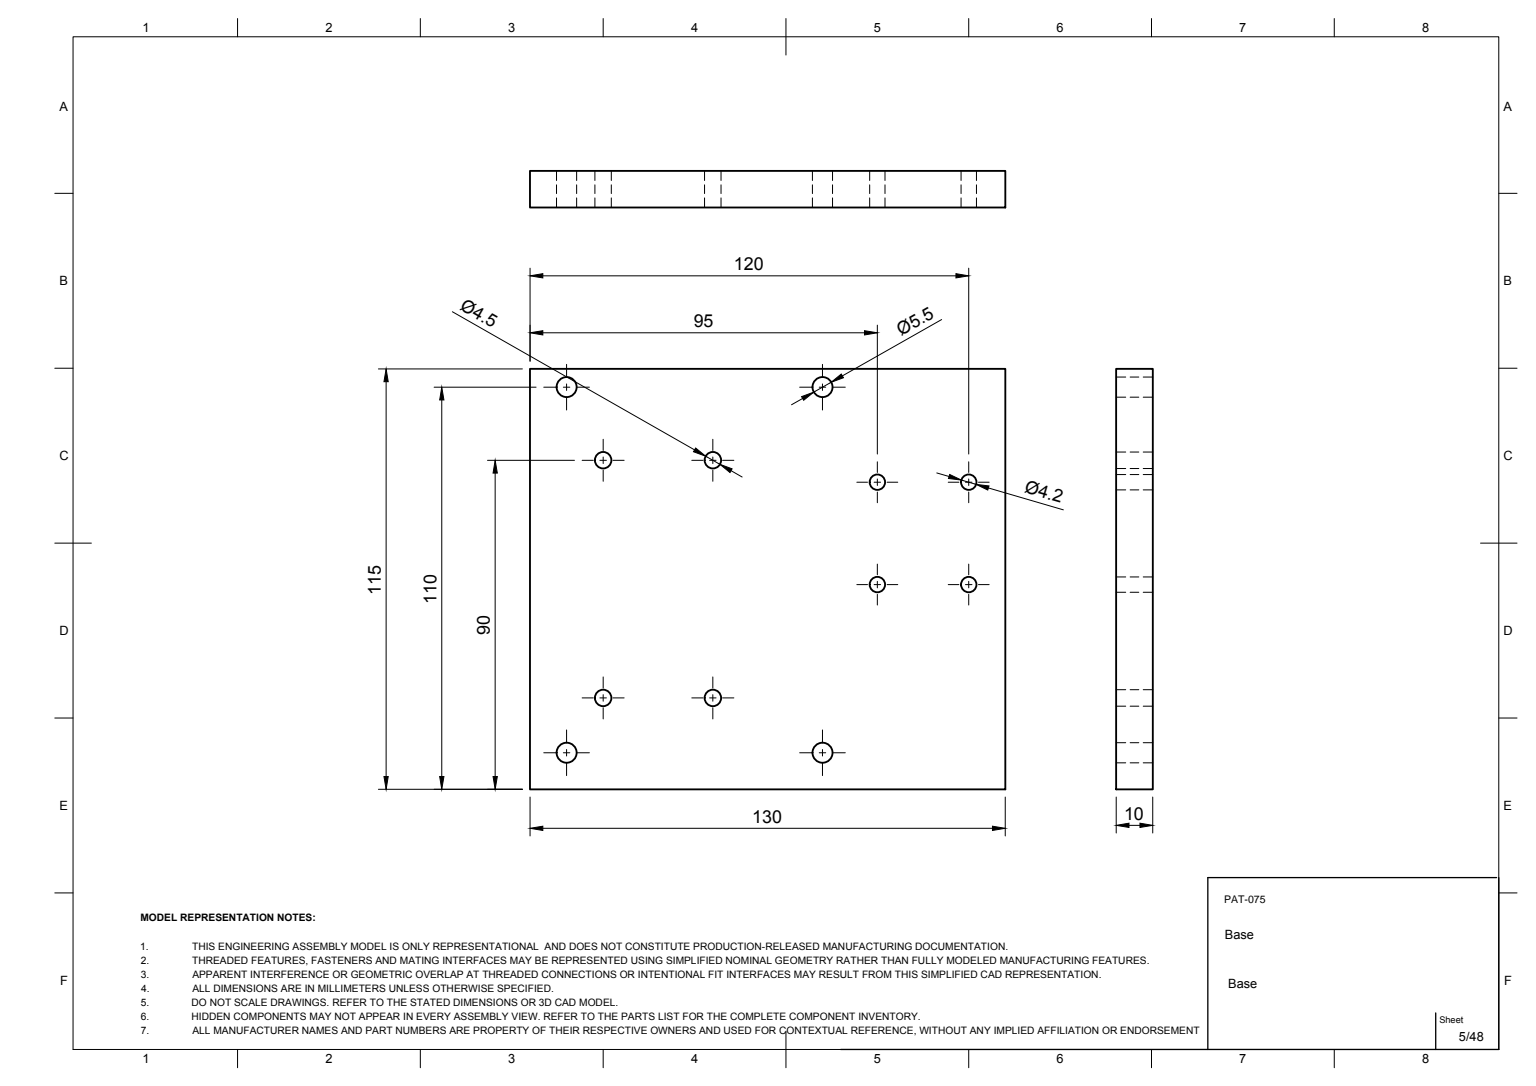
ISO-10303-21;
HEADER;
/* Generated by software containing ST-Developer
 * from STEP Tools, Inc. (www.steptools.com) 
 */

FILE_DESCRIPTION(
/* description */ ('Over-Centre Plunger Toggle Clamp on Slotted Fixture Frame'),
/* implementation_level */ '2;1');

FILE_NAME(
/* name */ 
'Base.step',
/* time_stamp */ '2026-10-28T03:23:24-07:00',
/* author */ (''),
/* organization */ (''),
/* preprocessor_version */ 'ST-DEVELOPER v20.2',
/* originating_system */ 'Autodesk Translation Framework v15.17.0.0',
/* authorisation */ '');

FILE_SCHEMA (('AUTOMOTIVE_DESIGN { 1 0 10303 214 3 1 1 }'));
ENDSEC;

DATA;
#10=MECHANICAL_DESIGN_GEOMETRIC_PRESENTATION_REPRESENTATION('',(#513),#15212);
#429=SHAPE_REPRESENTATION_RELATIONSHIP('SRR','None',#15403,#471);
#471=ADVANCED_BREP_SHAPE_REPRESENTATION('',(#564),#15165);
#513=STYLED_ITEM('',(#15698),#564);
#564=MANIFOLD_SOLID_BREP('Body1',#8245);
#611=FACE_BOUND('',#1590,.T.);
#612=FACE_BOUND('',#1591,.T.);
#613=FACE_BOUND('',#1592,.T.);
#614=FACE_BOUND('',#1593,.T.);
#615=FACE_BOUND('',#1594,.T.);
#616=FACE_BOUND('',#1595,.T.);
#617=FACE_BOUND('',#1596,.T.);
#618=FACE_BOUND('',#1597,.T.);
#619=FACE_BOUND('',#1598,.T.);
#620=FACE_BOUND('',#1599,.T.);
#621=FACE_BOUND('',#1600,.T.);
#622=FACE_BOUND('',#1601,.T.);
#623=FACE_BOUND('',#1603,.T.);
#624=FACE_BOUND('',#1604,.T.);
#625=FACE_BOUND('',#1605,.T.);
#626=FACE_BOUND('',#1606,.T.);
#627=FACE_BOUND('',#1607,.T.);
#628=FACE_BOUND('',#1608,.T.);
#629=FACE_BOUND('',#1609,.T.);
#630=FACE_BOUND('',#1610,.T.);
#631=FACE_BOUND('',#1611,.T.);
#632=FACE_BOUND('',#1612,.T.);
#633=FACE_BOUND('',#1613,.T.);
#634=FACE_BOUND('',#1614,.T.);
#783=PLANE('',#8802);
#784=PLANE('',#8803);
#785=PLANE('',#8804);
#786=PLANE('',#8805);
#787=PLANE('',#8806);
#788=PLANE('',#8807);
#1087=FACE_OUTER_BOUND('',#1573,.T.);
#1088=FACE_OUTER_BOUND('',#1574,.T.);
#1089=FACE_OUTER_BOUND('',#1575,.T.);
#1090=FACE_OUTER_BOUND('',#1576,.T.);
#1091=FACE_OUTER_BOUND('',#1577,.T.);
#1092=FACE_OUTER_BOUND('',#1578,.T.);
#1093=FACE_OUTER_BOUND('',#1579,.T.);
#1094=FACE_OUTER_BOUND('',#1580,.T.);
#1095=FACE_OUTER_BOUND('',#1581,.T.);
#1096=FACE_OUTER_BOUND('',#1582,.T.);
#1097=FACE_OUTER_BOUND('',#1583,.T.);
#1098=FACE_OUTER_BOUND('',#1584,.T.);
#1099=FACE_OUTER_BOUND('',#1585,.T.);
#1100=FACE_OUTER_BOUND('',#1586,.T.);
#1101=FACE_OUTER_BOUND('',#1587,.T.);
#1102=FACE_OUTER_BOUND('',#1588,.T.);
#1103=FACE_OUTER_BOUND('',#1589,.T.);
#1104=FACE_OUTER_BOUND('',#1602,.T.);
#1573=EDGE_LOOP('',(#5569,#5570,#5571,#5572));
#1574=EDGE_LOOP('',(#5573,#5574,#5575,#5576));
#1575=EDGE_LOOP('',(#5577,#5578,#5579,#5580));
#1576=EDGE_LOOP('',(#5581,#5582,#5583,#5584));
#1577=EDGE_LOOP('',(#5585,#5586,#5587,#5588));
#1578=EDGE_LOOP('',(#5589,#5590,#5591,#5592));
#1579=EDGE_LOOP('',(#5593,#5594,#5595,#5596));
#1580=EDGE_LOOP('',(#5597,#5598,#5599,#5600));
#1581=EDGE_LOOP('',(#5601,#5602,#5603,#5604));
#1582=EDGE_LOOP('',(#5605,#5606,#5607,#5608));
#1583=EDGE_LOOP('',(#5609,#5610,#5611,#5612));
#1584=EDGE_LOOP('',(#5613,#5614,#5615,#5616));
#1585=EDGE_LOOP('',(#5617,#5618,#5619,#5620));
#1586=EDGE_LOOP('',(#5621,#5622,#5623,#5624));
#1587=EDGE_LOOP('',(#5625,#5626,#5627,#5628));
#1588=EDGE_LOOP('',(#5629,#5630,#5631,#5632));
#1589=EDGE_LOOP('',(#5633,#5634,#5635,#5636));
#1590=EDGE_LOOP('',(#5637));
#1591=EDGE_LOOP('',(#5638));
#1592=EDGE_LOOP('',(#5639));
#1593=EDGE_LOOP('',(#5640));
#1594=EDGE_LOOP('',(#5641));
#1595=EDGE_LOOP('',(#5642));
#1596=EDGE_LOOP('',(#5643));
#1597=EDGE_LOOP('',(#5644));
#1598=EDGE_LOOP('',(#5645));
#1599=EDGE_LOOP('',(#5646));
#1600=EDGE_LOOP('',(#5647));
#1601=EDGE_LOOP('',(#5648));
#1602=EDGE_LOOP('',(#5649,#5650,#5651,#5652));
#1603=EDGE_LOOP('',(#5653));
#1604=EDGE_LOOP('',(#5654));
#1605=EDGE_LOOP('',(#5655));
#1606=EDGE_LOOP('',(#5656));
#1607=EDGE_LOOP('',(#5657));
#1608=EDGE_LOOP('',(#5658));
#1609=EDGE_LOOP('',(#5659));
#1610=EDGE_LOOP('',(#5660));
#1611=EDGE_LOOP('',(#5661));
#1612=EDGE_LOOP('',(#5662));
#1613=EDGE_LOOP('',(#5663));
#1614=EDGE_LOOP('',(#5664));
#2231=LINE('',#12373,#2861);
#2232=LINE('',#12379,#2862);
#2233=LINE('',#12385,#2863);
#2234=LINE('',#12391,#2864);
#2235=LINE('',#12397,#2865);
#2236=LINE('',#12403,#2866);
#2237=LINE('',#12409,#2867);
#2238=LINE('',#12415,#2868);
#2239=LINE('',#12421,#2869);
#2240=LINE('',#12427,#2870);
#2241=LINE('',#12433,#2871);
#2242=LINE('',#12439,#2872);
#2243=LINE('',#12444,#2873);
#2244=LINE('',#12446,#2874);
#2245=LINE('',#12448,#2875);
#2246=LINE('',#12449,#2876);
#2247=LINE('',#12452,#2877);
#2248=LINE('',#12454,#2878);
#2249=LINE('',#12455,#2879);
#2250=LINE('',#12458,#2880);
#2251=LINE('',#12460,#2881);
#2252=LINE('',#12461,#2882);
#2253=LINE('',#12463,#2883);
#2254=LINE('',#12464,#2884);
#2861=VECTOR('',#9764,0.225);
#2862=VECTOR('',#9771,0.225);
#2863=VECTOR('',#9778,0.225);
#2864=VECTOR('',#9785,0.225);
#2865=VECTOR('',#9792,0.21);
#2866=VECTOR('',#9799,0.210000000000001);
#2867=VECTOR('',#9806,0.210000000000001);
#2868=VECTOR('',#9813,0.21);
#2869=VECTOR('',#9820,0.275);
#2870=VECTOR('',#9827,0.275);
#2871=VECTOR('',#9834,0.275);
#2872=VECTOR('',#9841,0.275);
#2873=VECTOR('',#9846,1.);
#2874=VECTOR('',#9847,1.);
#2875=VECTOR('',#9848,1.);
#2876=VECTOR('',#9849,1.);
#2877=VECTOR('',#9852,1.);
#2878=VECTOR('',#9853,1.);
#2879=VECTOR('',#9854,1.);
#2880=VECTOR('',#9857,1.);
#2881=VECTOR('',#9858,1.);
#2882=VECTOR('',#9859,1.);
#2883=VECTOR('',#9862,1.);
#2884=VECTOR('',#9863,1.);
#3491=CIRCLE('',#8767,0.225);
#3492=CIRCLE('',#8768,0.225);
#3493=CIRCLE('',#8770,0.225);
#3494=CIRCLE('',#8771,0.225);
#3495=CIRCLE('',#8773,0.225);
#3496=CIRCLE('',#8774,0.225);
#3497=CIRCLE('',#8776,0.225);
#3498=CIRCLE('',#8777,0.225);
#3499=CIRCLE('',#8779,0.21);
#3500=CIRCLE('',#8780,0.21);
#3501=CIRCLE('',#8782,0.210000000000001);
#3502=CIRCLE('',#8783,0.210000000000001);
#3503=CIRCLE('',#8785,0.210000000000001);
#3504=CIRCLE('',#8786,0.210000000000001);
#3505=CIRCLE('',#8788,0.21);
#3506=CIRCLE('',#8789,0.21);
#3507=CIRCLE('',#8791,0.275);
#3508=CIRCLE('',#8792,0.275);
#3509=CIRCLE('',#8794,0.275);
#3510=CIRCLE('',#8795,0.275);
#3511=CIRCLE('',#8797,0.275);
#3512=CIRCLE('',#8798,0.275);
#3513=CIRCLE('',#8800,0.275);
#3514=CIRCLE('',#8801,0.275);
#3859=VERTEX_POINT('',#12370);
#3860=VERTEX_POINT('',#12372);
#3861=VERTEX_POINT('',#12376);
#3862=VERTEX_POINT('',#12378);
#3863=VERTEX_POINT('',#12382);
#3864=VERTEX_POINT('',#12384);
#3865=VERTEX_POINT('',#12388);
#3866=VERTEX_POINT('',#12390);
#3867=VERTEX_POINT('',#12394);
#3868=VERTEX_POINT('',#12396);
#3869=VERTEX_POINT('',#12400);
#3870=VERTEX_POINT('',#12402);
#3871=VERTEX_POINT('',#12406);
#3872=VERTEX_POINT('',#12408);
#3873=VERTEX_POINT('',#12412);
#3874=VERTEX_POINT('',#12414);
#3875=VERTEX_POINT('',#12418);
#3876=VERTEX_POINT('',#12420);
#3877=VERTEX_POINT('',#12424);
#3878=VERTEX_POINT('',#12426);
#3879=VERTEX_POINT('',#12430);
#3880=VERTEX_POINT('',#12432);
#3881=VERTEX_POINT('',#12436);
#3882=VERTEX_POINT('',#12438);
#3883=VERTEX_POINT('',#12442);
#3884=VERTEX_POINT('',#12443);
#3885=VERTEX_POINT('',#12445);
#3886=VERTEX_POINT('',#12447);
#3887=VERTEX_POINT('',#12451);
#3888=VERTEX_POINT('',#12453);
#3889=VERTEX_POINT('',#12457);
#3890=VERTEX_POINT('',#12459);
#4545=EDGE_CURVE('',#3859,#3859,#3491,.T.);
#4546=EDGE_CURVE('',#3859,#3860,#2231,.T.);
#4547=EDGE_CURVE('',#3860,#3860,#3492,.T.);
#4548=EDGE_CURVE('',#3861,#3861,#3493,.T.);
#4549=EDGE_CURVE('',#3861,#3862,#2232,.T.);
#4550=EDGE_CURVE('',#3862,#3862,#3494,.T.);
#4551=EDGE_CURVE('',#3863,#3863,#3495,.T.);
#4552=EDGE_CURVE('',#3863,#3864,#2233,.T.);
#4553=EDGE_CURVE('',#3864,#3864,#3496,.T.);
#4554=EDGE_CURVE('',#3865,#3865,#3497,.T.);
#4555=EDGE_CURVE('',#3865,#3866,#2234,.T.);
#4556=EDGE_CURVE('',#3866,#3866,#3498,.T.);
#4557=EDGE_CURVE('',#3867,#3867,#3499,.T.);
#4558=EDGE_CURVE('',#3867,#3868,#2235,.T.);
#4559=EDGE_CURVE('',#3868,#3868,#3500,.T.);
#4560=EDGE_CURVE('',#3869,#3869,#3501,.T.);
#4561=EDGE_CURVE('',#3869,#3870,#2236,.T.);
#4562=EDGE_CURVE('',#3870,#3870,#3502,.T.);
#4563=EDGE_CURVE('',#3871,#3871,#3503,.T.);
#4564=EDGE_CURVE('',#3871,#3872,#2237,.T.);
#4565=EDGE_CURVE('',#3872,#3872,#3504,.T.);
#4566=EDGE_CURVE('',#3873,#3873,#3505,.T.);
#4567=EDGE_CURVE('',#3873,#3874,#2238,.T.);
#4568=EDGE_CURVE('',#3874,#3874,#3506,.T.);
#4569=EDGE_CURVE('',#3875,#3875,#3507,.T.);
#4570=EDGE_CURVE('',#3875,#3876,#2239,.T.);
#4571=EDGE_CURVE('',#3876,#3876,#3508,.T.);
#4572=EDGE_CURVE('',#3877,#3877,#3509,.T.);
#4573=EDGE_CURVE('',#3877,#3878,#2240,.T.);
#4574=EDGE_CURVE('',#3878,#3878,#3510,.T.);
#4575=EDGE_CURVE('',#3879,#3879,#3511,.T.);
#4576=EDGE_CURVE('',#3879,#3880,#2241,.T.);
#4577=EDGE_CURVE('',#3880,#3880,#3512,.T.);
#4578=EDGE_CURVE('',#3881,#3881,#3513,.T.);
#4579=EDGE_CURVE('',#3881,#3882,#2242,.T.);
#4580=EDGE_CURVE('',#3882,#3882,#3514,.T.);
#4581=EDGE_CURVE('',#3883,#3884,#2243,.T.);
#4582=EDGE_CURVE('',#3884,#3885,#2244,.T.);
#4583=EDGE_CURVE('',#3886,#3885,#2245,.T.);
#4584=EDGE_CURVE('',#3883,#3886,#2246,.T.);
#4585=EDGE_CURVE('',#3887,#3883,#2247,.T.);
#4586=EDGE_CURVE('',#3888,#3886,#2248,.T.);
#4587=EDGE_CURVE('',#3887,#3888,#2249,.T.);
#4588=EDGE_CURVE('',#3889,#3887,#2250,.T.);
#4589=EDGE_CURVE('',#3890,#3888,#2251,.T.);
#4590=EDGE_CURVE('',#3889,#3890,#2252,.T.);
#4591=EDGE_CURVE('',#3884,#3889,#2253,.T.);
#4592=EDGE_CURVE('',#3885,#3890,#2254,.T.);
#5569=ORIENTED_EDGE('',*,*,#4545,.F.);
#5570=ORIENTED_EDGE('',*,*,#4546,.T.);
#5571=ORIENTED_EDGE('',*,*,#4547,.F.);
#5572=ORIENTED_EDGE('',*,*,#4546,.F.);
#5573=ORIENTED_EDGE('',*,*,#4548,.F.);
#5574=ORIENTED_EDGE('',*,*,#4549,.T.);
#5575=ORIENTED_EDGE('',*,*,#4550,.F.);
#5576=ORIENTED_EDGE('',*,*,#4549,.F.);
#5577=ORIENTED_EDGE('',*,*,#4551,.F.);
#5578=ORIENTED_EDGE('',*,*,#4552,.T.);
#5579=ORIENTED_EDGE('',*,*,#4553,.F.);
#5580=ORIENTED_EDGE('',*,*,#4552,.F.);
#5581=ORIENTED_EDGE('',*,*,#4554,.F.);
#5582=ORIENTED_EDGE('',*,*,#4555,.T.);
#5583=ORIENTED_EDGE('',*,*,#4556,.F.);
#5584=ORIENTED_EDGE('',*,*,#4555,.F.);
#5585=ORIENTED_EDGE('',*,*,#4557,.F.);
#5586=ORIENTED_EDGE('',*,*,#4558,.T.);
#5587=ORIENTED_EDGE('',*,*,#4559,.F.);
#5588=ORIENTED_EDGE('',*,*,#4558,.F.);
#5589=ORIENTED_EDGE('',*,*,#4560,.F.);
#5590=ORIENTED_EDGE('',*,*,#4561,.T.);
#5591=ORIENTED_EDGE('',*,*,#4562,.F.);
#5592=ORIENTED_EDGE('',*,*,#4561,.F.);
#5593=ORIENTED_EDGE('',*,*,#4563,.F.);
#5594=ORIENTED_EDGE('',*,*,#4564,.T.);
#5595=ORIENTED_EDGE('',*,*,#4565,.F.);
#5596=ORIENTED_EDGE('',*,*,#4564,.F.);
#5597=ORIENTED_EDGE('',*,*,#4566,.F.);
#5598=ORIENTED_EDGE('',*,*,#4567,.T.);
#5599=ORIENTED_EDGE('',*,*,#4568,.F.);
#5600=ORIENTED_EDGE('',*,*,#4567,.F.);
#5601=ORIENTED_EDGE('',*,*,#4569,.F.);
#5602=ORIENTED_EDGE('',*,*,#4570,.T.);
#5603=ORIENTED_EDGE('',*,*,#4571,.F.);
#5604=ORIENTED_EDGE('',*,*,#4570,.F.);
#5605=ORIENTED_EDGE('',*,*,#4572,.F.);
#5606=ORIENTED_EDGE('',*,*,#4573,.T.);
#5607=ORIENTED_EDGE('',*,*,#4574,.F.);
#5608=ORIENTED_EDGE('',*,*,#4573,.F.);
#5609=ORIENTED_EDGE('',*,*,#4575,.F.);
#5610=ORIENTED_EDGE('',*,*,#4576,.T.);
#5611=ORIENTED_EDGE('',*,*,#4577,.F.);
#5612=ORIENTED_EDGE('',*,*,#4576,.F.);
#5613=ORIENTED_EDGE('',*,*,#4578,.F.);
#5614=ORIENTED_EDGE('',*,*,#4579,.T.);
#5615=ORIENTED_EDGE('',*,*,#4580,.F.);
#5616=ORIENTED_EDGE('',*,*,#4579,.F.);
#5617=ORIENTED_EDGE('',*,*,#4581,.T.);
#5618=ORIENTED_EDGE('',*,*,#4582,.T.);
#5619=ORIENTED_EDGE('',*,*,#4583,.F.);
#5620=ORIENTED_EDGE('',*,*,#4584,.F.);
#5621=ORIENTED_EDGE('',*,*,#4585,.T.);
#5622=ORIENTED_EDGE('',*,*,#4584,.T.);
#5623=ORIENTED_EDGE('',*,*,#4586,.F.);
#5624=ORIENTED_EDGE('',*,*,#4587,.F.);
#5625=ORIENTED_EDGE('',*,*,#4588,.T.);
#5626=ORIENTED_EDGE('',*,*,#4587,.T.);
#5627=ORIENTED_EDGE('',*,*,#4589,.F.);
#5628=ORIENTED_EDGE('',*,*,#4590,.F.);
#5629=ORIENTED_EDGE('',*,*,#4591,.T.);
#5630=ORIENTED_EDGE('',*,*,#4590,.T.);
#5631=ORIENTED_EDGE('',*,*,#4592,.F.);
#5632=ORIENTED_EDGE('',*,*,#4582,.F.);
#5633=ORIENTED_EDGE('',*,*,#4592,.T.);
#5634=ORIENTED_EDGE('',*,*,#4589,.T.);
#5635=ORIENTED_EDGE('',*,*,#4586,.T.);
#5636=ORIENTED_EDGE('',*,*,#4583,.T.);
#5637=ORIENTED_EDGE('',*,*,#4553,.T.);
#5638=ORIENTED_EDGE('',*,*,#4556,.T.);
#5639=ORIENTED_EDGE('',*,*,#4580,.T.);
#5640=ORIENTED_EDGE('',*,*,#4577,.T.);
#5641=ORIENTED_EDGE('',*,*,#4574,.T.);
#5642=ORIENTED_EDGE('',*,*,#4571,.T.);
#5643=ORIENTED_EDGE('',*,*,#4568,.T.);
#5644=ORIENTED_EDGE('',*,*,#4565,.T.);
#5645=ORIENTED_EDGE('',*,*,#4562,.T.);
#5646=ORIENTED_EDGE('',*,*,#4559,.T.);
#5647=ORIENTED_EDGE('',*,*,#4550,.T.);
#5648=ORIENTED_EDGE('',*,*,#4547,.T.);
#5649=ORIENTED_EDGE('',*,*,#4591,.F.);
#5650=ORIENTED_EDGE('',*,*,#4581,.F.);
#5651=ORIENTED_EDGE('',*,*,#4585,.F.);
#5652=ORIENTED_EDGE('',*,*,#4588,.F.);
#5653=ORIENTED_EDGE('',*,*,#4551,.T.);
#5654=ORIENTED_EDGE('',*,*,#4554,.T.);
#5655=ORIENTED_EDGE('',*,*,#4578,.T.);
#5656=ORIENTED_EDGE('',*,*,#4575,.T.);
#5657=ORIENTED_EDGE('',*,*,#4572,.T.);
#5658=ORIENTED_EDGE('',*,*,#4569,.T.);
#5659=ORIENTED_EDGE('',*,*,#4566,.T.);
#5660=ORIENTED_EDGE('',*,*,#4563,.T.);
#5661=ORIENTED_EDGE('',*,*,#4560,.T.);
#5662=ORIENTED_EDGE('',*,*,#4557,.T.);
#5663=ORIENTED_EDGE('',*,*,#4548,.T.);
#5664=ORIENTED_EDGE('',*,*,#4545,.T.);
#7617=CYLINDRICAL_SURFACE('',#8766,0.225);
#7618=CYLINDRICAL_SURFACE('',#8769,0.225);
#7619=CYLINDRICAL_SURFACE('',#8772,0.225);
#7620=CYLINDRICAL_SURFACE('',#8775,0.225);
#7621=CYLINDRICAL_SURFACE('',#8778,0.21);
#7622=CYLINDRICAL_SURFACE('',#8781,0.210000000000001);
#7623=CYLINDRICAL_SURFACE('',#8784,0.210000000000001);
#7624=CYLINDRICAL_SURFACE('',#8787,0.21);
#7625=CYLINDRICAL_SURFACE('',#8790,0.275);
#7626=CYLINDRICAL_SURFACE('',#8793,0.275);
#7627=CYLINDRICAL_SURFACE('',#8796,0.275);
#7628=CYLINDRICAL_SURFACE('',#8799,0.275);
#7759=ADVANCED_FACE('',(#1087),#7617,.F.);
#7760=ADVANCED_FACE('',(#1088),#7618,.F.);
#7761=ADVANCED_FACE('',(#1089),#7619,.F.);
#7762=ADVANCED_FACE('',(#1090),#7620,.F.);
#7763=ADVANCED_FACE('',(#1091),#7621,.F.);
#7764=ADVANCED_FACE('',(#1092),#7622,.F.);
#7765=ADVANCED_FACE('',(#1093),#7623,.F.);
#7766=ADVANCED_FACE('',(#1094),#7624,.F.);
#7767=ADVANCED_FACE('',(#1095),#7625,.F.);
#7768=ADVANCED_FACE('',(#1096),#7626,.F.);
#7769=ADVANCED_FACE('',(#1097),#7627,.F.);
#7770=ADVANCED_FACE('',(#1098),#7628,.F.);
#7771=ADVANCED_FACE('',(#1099),#783,.T.);
#7772=ADVANCED_FACE('',(#1100),#784,.T.);
#7773=ADVANCED_FACE('',(#1101),#785,.T.);
#7774=ADVANCED_FACE('',(#1102),#786,.T.);
#7775=ADVANCED_FACE('',(#1103,#611,#612,#613,#614,#615,#616,#617,#618,#619,
#620,#621,#622),#787,.T.);
#7776=ADVANCED_FACE('',(#1104,#623,#624,#625,#626,#627,#628,#629,#630,#631,
#632,#633,#634),#788,.F.);
#8245=CLOSED_SHELL('',(#7759,#7760,#7761,#7762,#7763,#7764,#7765,#7766,
#7767,#7768,#7769,#7770,#7771,#7772,#7773,#7774,#7775,#7776));
#8765=AXIS2_PLACEMENT_3D('',#12368,#9758,#9759);
#8766=AXIS2_PLACEMENT_3D('',#12369,#9760,#9761);
#8767=AXIS2_PLACEMENT_3D('',#12371,#9762,#9763);
#8768=AXIS2_PLACEMENT_3D('',#12374,#9765,#9766);
#8769=AXIS2_PLACEMENT_3D('',#12375,#9767,#9768);
#8770=AXIS2_PLACEMENT_3D('',#12377,#9769,#9770);
#8771=AXIS2_PLACEMENT_3D('',#12380,#9772,#9773);
#8772=AXIS2_PLACEMENT_3D('',#12381,#9774,#9775);
#8773=AXIS2_PLACEMENT_3D('',#12383,#9776,#9777);
#8774=AXIS2_PLACEMENT_3D('',#12386,#9779,#9780);
#8775=AXIS2_PLACEMENT_3D('',#12387,#9781,#9782);
#8776=AXIS2_PLACEMENT_3D('',#12389,#9783,#9784);
#8777=AXIS2_PLACEMENT_3D('',#12392,#9786,#9787);
#8778=AXIS2_PLACEMENT_3D('',#12393,#9788,#9789);
#8779=AXIS2_PLACEMENT_3D('',#12395,#9790,#9791);
#8780=AXIS2_PLACEMENT_3D('',#12398,#9793,#9794);
#8781=AXIS2_PLACEMENT_3D('',#12399,#9795,#9796);
#8782=AXIS2_PLACEMENT_3D('',#12401,#9797,#9798);
#8783=AXIS2_PLACEMENT_3D('',#12404,#9800,#9801);
#8784=AXIS2_PLACEMENT_3D('',#12405,#9802,#9803);
#8785=AXIS2_PLACEMENT_3D('',#12407,#9804,#9805);
#8786=AXIS2_PLACEMENT_3D('',#12410,#9807,#9808);
#8787=AXIS2_PLACEMENT_3D('',#12411,#9809,#9810);
#8788=AXIS2_PLACEMENT_3D('',#12413,#9811,#9812);
#8789=AXIS2_PLACEMENT_3D('',#12416,#9814,#9815);
#8790=AXIS2_PLACEMENT_3D('',#12417,#9816,#9817);
#8791=AXIS2_PLACEMENT_3D('',#12419,#9818,#9819);
#8792=AXIS2_PLACEMENT_3D('',#12422,#9821,#9822);
#8793=AXIS2_PLACEMENT_3D('',#12423,#9823,#9824);
#8794=AXIS2_PLACEMENT_3D('',#12425,#9825,#9826);
#8795=AXIS2_PLACEMENT_3D('',#12428,#9828,#9829);
#8796=AXIS2_PLACEMENT_3D('',#12429,#9830,#9831);
#8797=AXIS2_PLACEMENT_3D('',#12431,#9832,#9833);
#8798=AXIS2_PLACEMENT_3D('',#12434,#9835,#9836);
#8799=AXIS2_PLACEMENT_3D('',#12435,#9837,#9838);
#8800=AXIS2_PLACEMENT_3D('',#12437,#9839,#9840);
#8801=AXIS2_PLACEMENT_3D('',#12440,#9842,#9843);
#8802=AXIS2_PLACEMENT_3D('',#12441,#9844,#9845);
#8803=AXIS2_PLACEMENT_3D('',#12450,#9850,#9851);
#8804=AXIS2_PLACEMENT_3D('',#12456,#9855,#9856);
#8805=AXIS2_PLACEMENT_3D('',#12462,#9860,#9861);
#8806=AXIS2_PLACEMENT_3D('',#12465,#9864,#9865);
#8807=AXIS2_PLACEMENT_3D('',#12466,#9866,#9867);
#9758=DIRECTION('axis',(0.,0.,1.));
#9759=DIRECTION('refdir',(1.,0.,0.));
#9760=DIRECTION('center_axis',(0.,0.,1.));
#9761=DIRECTION('ref_axis',(1.,0.,0.));
#9762=DIRECTION('center_axis',(0.,0.,1.));
#9763=DIRECTION('ref_axis',(1.,0.,0.));
#9764=DIRECTION('',(0.,0.,1.));
#9765=DIRECTION('center_axis',(0.,0.,-1.));
#9766=DIRECTION('ref_axis',(1.,0.,0.));
#9767=DIRECTION('center_axis',(0.,0.,1.));
#9768=DIRECTION('ref_axis',(1.,0.,0.));
#9769=DIRECTION('center_axis',(0.,0.,1.));
#9770=DIRECTION('ref_axis',(1.,0.,0.));
#9771=DIRECTION('',(0.,0.,1.));
#9772=DIRECTION('center_axis',(0.,0.,-1.));
#9773=DIRECTION('ref_axis',(1.,0.,0.));
#9774=DIRECTION('center_axis',(0.,0.,1.));
#9775=DIRECTION('ref_axis',(1.,0.,0.));
#9776=DIRECTION('center_axis',(0.,0.,1.));
#9777=DIRECTION('ref_axis',(1.,0.,0.));
#9778=DIRECTION('',(0.,0.,1.));
#9779=DIRECTION('center_axis',(0.,0.,-1.));
#9780=DIRECTION('ref_axis',(1.,0.,0.));
#9781=DIRECTION('center_axis',(0.,0.,1.));
#9782=DIRECTION('ref_axis',(1.,0.,0.));
#9783=DIRECTION('center_axis',(0.,0.,1.));
#9784=DIRECTION('ref_axis',(1.,0.,0.));
#9785=DIRECTION('',(0.,0.,1.));
#9786=DIRECTION('center_axis',(0.,0.,-1.));
#9787=DIRECTION('ref_axis',(1.,0.,0.));
#9788=DIRECTION('center_axis',(0.,0.,1.));
#9789=DIRECTION('ref_axis',(1.,0.,0.));
#9790=DIRECTION('center_axis',(0.,0.,1.));
#9791=DIRECTION('ref_axis',(1.,0.,0.));
#9792=DIRECTION('',(0.,0.,1.));
#9793=DIRECTION('center_axis',(0.,0.,-1.));
#9794=DIRECTION('ref_axis',(1.,0.,0.));
#9795=DIRECTION('center_axis',(0.,0.,1.));
#9796=DIRECTION('ref_axis',(1.,0.,0.));
#9797=DIRECTION('center_axis',(0.,0.,1.));
#9798=DIRECTION('ref_axis',(1.,0.,0.));
#9799=DIRECTION('',(0.,0.,1.));
#9800=DIRECTION('center_axis',(0.,0.,-1.));
#9801=DIRECTION('ref_axis',(1.,0.,0.));
#9802=DIRECTION('center_axis',(0.,0.,1.));
#9803=DIRECTION('ref_axis',(1.,0.,0.));
#9804=DIRECTION('center_axis',(0.,0.,1.));
#9805=DIRECTION('ref_axis',(1.,0.,0.));
#9806=DIRECTION('',(0.,0.,1.));
#9807=DIRECTION('center_axis',(0.,0.,-1.));
#9808=DIRECTION('ref_axis',(1.,0.,0.));
#9809=DIRECTION('center_axis',(0.,0.,1.));
#9810=DIRECTION('ref_axis',(1.,0.,0.));
#9811=DIRECTION('center_axis',(0.,0.,1.));
#9812=DIRECTION('ref_axis',(1.,0.,0.));
#9813=DIRECTION('',(0.,0.,1.));
#9814=DIRECTION('center_axis',(0.,0.,-1.));
#9815=DIRECTION('ref_axis',(1.,0.,0.));
#9816=DIRECTION('center_axis',(0.,0.,1.));
#9817=DIRECTION('ref_axis',(1.,0.,0.));
#9818=DIRECTION('center_axis',(0.,0.,1.));
#9819=DIRECTION('ref_axis',(1.,0.,0.));
#9820=DIRECTION('',(0.,0.,1.));
#9821=DIRECTION('center_axis',(0.,0.,-1.));
#9822=DIRECTION('ref_axis',(1.,0.,0.));
#9823=DIRECTION('center_axis',(0.,0.,1.));
#9824=DIRECTION('ref_axis',(1.,0.,0.));
#9825=DIRECTION('center_axis',(0.,0.,1.));
#9826=DIRECTION('ref_axis',(1.,0.,0.));
#9827=DIRECTION('',(0.,0.,1.));
#9828=DIRECTION('center_axis',(0.,0.,-1.));
#9829=DIRECTION('ref_axis',(1.,0.,0.));
#9830=DIRECTION('center_axis',(0.,0.,1.));
#9831=DIRECTION('ref_axis',(1.,0.,0.));
#9832=DIRECTION('center_axis',(0.,0.,1.));
#9833=DIRECTION('ref_axis',(1.,0.,0.));
#9834=DIRECTION('',(0.,0.,1.));
#9835=DIRECTION('center_axis',(0.,0.,-1.));
#9836=DIRECTION('ref_axis',(1.,0.,0.));
#9837=DIRECTION('center_axis',(0.,0.,1.));
#9838=DIRECTION('ref_axis',(1.,0.,0.));
#9839=DIRECTION('center_axis',(0.,0.,1.));
#9840=DIRECTION('ref_axis',(1.,0.,0.));
#9841=DIRECTION('',(0.,0.,1.));
#9842=DIRECTION('center_axis',(0.,0.,-1.));
#9843=DIRECTION('ref_axis',(1.,0.,0.));
#9844=DIRECTION('center_axis',(0.,1.,0.));
#9845=DIRECTION('ref_axis',(-1.,0.,0.));
#9846=DIRECTION('',(-1.,0.,0.));
#9847=DIRECTION('',(0.,0.,1.));
#9848=DIRECTION('',(-1.,0.,0.));
#9849=DIRECTION('',(0.,0.,1.));
#9850=DIRECTION('center_axis',(1.,0.,0.));
#9851=DIRECTION('ref_axis',(0.,1.,0.));
#9852=DIRECTION('',(0.,1.,0.));
#9853=DIRECTION('',(0.,1.,0.));
#9854=DIRECTION('',(0.,0.,1.));
#9855=DIRECTION('center_axis',(0.,-1.,0.));
#9856=DIRECTION('ref_axis',(1.,0.,0.));
#9857=DIRECTION('',(1.,0.,0.));
#9858=DIRECTION('',(1.,0.,0.));
#9859=DIRECTION('',(0.,0.,1.));
#9860=DIRECTION('center_axis',(-1.,0.,0.));
#9861=DIRECTION('ref_axis',(0.,-1.,0.));
#9862=DIRECTION('',(0.,-1.,0.));
#9863=DIRECTION('',(0.,-1.,0.));
#9864=DIRECTION('center_axis',(0.,0.,1.));
#9865=DIRECTION('ref_axis',(1.,0.,0.));
#9866=DIRECTION('center_axis',(0.,0.,1.));
#9867=DIRECTION('ref_axis',(1.,0.,0.));
#12368=CARTESIAN_POINT('',(0.,0.,0.));
#12369=CARTESIAN_POINT('Origin',(1.5,-4.5,-0.1));
#12370=CARTESIAN_POINT('',(1.275,-4.5,0.));
#12371=CARTESIAN_POINT('Origin',(1.5,-4.5,0.));
#12372=CARTESIAN_POINT('',(1.275,-4.5,1.));
#12373=CARTESIAN_POINT('',(1.275,-4.5,-0.1));
#12374=CARTESIAN_POINT('Origin',(1.5,-4.5,1.));
#12375=CARTESIAN_POINT('Origin',(1.5,2.,-0.1));
#12376=CARTESIAN_POINT('',(1.275,2.,0.));
#12377=CARTESIAN_POINT('Origin',(1.5,2.,0.));
#12378=CARTESIAN_POINT('',(1.275,2.,1.));
#12379=CARTESIAN_POINT('',(1.275,2.,-0.1));
#12380=CARTESIAN_POINT('Origin',(1.5,2.,1.));
#12381=CARTESIAN_POINT('Origin',(-1.5,-4.5,-0.1));
#12382=CARTESIAN_POINT('',(-1.725,-4.5,0.));
#12383=CARTESIAN_POINT('Origin',(-1.5,-4.5,0.));
#12384=CARTESIAN_POINT('',(-1.725,-4.5,1.));
#12385=CARTESIAN_POINT('',(-1.725,-4.5,-0.1));
#12386=CARTESIAN_POINT('Origin',(-1.5,-4.5,1.));
#12387=CARTESIAN_POINT('Origin',(-1.5,2.,-0.1));
#12388=CARTESIAN_POINT('',(-1.725,2.,0.));
#12389=CARTESIAN_POINT('Origin',(-1.5,2.,0.));
#12390=CARTESIAN_POINT('',(-1.725,2.,1.));
#12391=CARTESIAN_POINT('',(-1.725,2.,-0.1));
#12392=CARTESIAN_POINT('Origin',(-1.5,2.,1.));
#12393=CARTESIAN_POINT('Origin',(-6.,-1.4,-0.1));
#12394=CARTESIAN_POINT('',(-6.21,-1.4,0.));
#12395=CARTESIAN_POINT('Origin',(-6.,-1.4,0.));
#12396=CARTESIAN_POINT('',(-6.21,-1.4,1.));
#12397=CARTESIAN_POINT('',(-6.21,-1.4,-0.1));
#12398=CARTESIAN_POINT('Origin',(-6.,-1.4,1.));
#12399=CARTESIAN_POINT('Origin',(-8.5,1.4,-0.1));
#12400=CARTESIAN_POINT('',(-8.71,1.4,0.));
#12401=CARTESIAN_POINT('Origin',(-8.5,1.4,0.));
#12402=CARTESIAN_POINT('',(-8.71,1.4,1.));
#12403=CARTESIAN_POINT('',(-8.71,1.4,-0.1));
#12404=CARTESIAN_POINT('Origin',(-8.5,1.4,1.));
#12405=CARTESIAN_POINT('Origin',(-8.5,-1.4,-0.1));
#12406=CARTESIAN_POINT('',(-8.71,-1.4,0.));
#12407=CARTESIAN_POINT('Origin',(-8.5,-1.4,0.));
#12408=CARTESIAN_POINT('',(-8.71,-1.4,1.));
#12409=CARTESIAN_POINT('',(-8.71,-1.4,-0.1));
#12410=CARTESIAN_POINT('Origin',(-8.5,-1.4,1.));
#12411=CARTESIAN_POINT('Origin',(-6.,1.4,-0.1));
#12412=CARTESIAN_POINT('',(-6.21,1.4,0.));
#12413=CARTESIAN_POINT('Origin',(-6.,1.4,0.));
#12414=CARTESIAN_POINT('',(-6.21,1.4,1.));
#12415=CARTESIAN_POINT('',(-6.21,1.4,-0.1));
#12416=CARTESIAN_POINT('Origin',(-6.,1.4,1.));
#12417=CARTESIAN_POINT('Origin',(2.5,4.,-0.1));
#12418=CARTESIAN_POINT('',(2.225,4.,0.));
#12419=CARTESIAN_POINT('Origin',(2.5,4.,0.));
#12420=CARTESIAN_POINT('',(2.225,4.,1.));
#12421=CARTESIAN_POINT('',(2.225,4.,-0.1));
#12422=CARTESIAN_POINT('Origin',(2.5,4.,1.));
#12423=CARTESIAN_POINT('Origin',(-4.5,4.,-0.1));
#12424=CARTESIAN_POINT('',(-4.775,4.,0.));
#12425=CARTESIAN_POINT('Origin',(-4.5,4.,0.));
#12426=CARTESIAN_POINT('',(-4.775,4.,1.));
#12427=CARTESIAN_POINT('',(-4.775,4.,-0.1));
#12428=CARTESIAN_POINT('Origin',(-4.5,4.,1.));
#12429=CARTESIAN_POINT('Origin',(2.5,-6.,-0.1));
#12430=CARTESIAN_POINT('',(2.225,-6.,0.));
#12431=CARTESIAN_POINT('Origin',(2.5,-6.,0.));
#12432=CARTESIAN_POINT('',(2.225,-6.,1.));
#12433=CARTESIAN_POINT('',(2.225,-6.,-0.1));
#12434=CARTESIAN_POINT('Origin',(2.5,-6.,1.));
#12435=CARTESIAN_POINT('Origin',(-4.5,-6.,-0.1));
#12436=CARTESIAN_POINT('',(-4.775,-6.,0.));
#12437=CARTESIAN_POINT('Origin',(-4.5,-6.,0.));
#12438=CARTESIAN_POINT('',(-4.775,-6.,1.));
#12439=CARTESIAN_POINT('',(-4.775,-6.,-0.1));
#12440=CARTESIAN_POINT('Origin',(-4.5,-6.,1.));
#12441=CARTESIAN_POINT('Origin',(3.5,4.5,0.));
#12442=CARTESIAN_POINT('',(3.5,4.5,0.));
#12443=CARTESIAN_POINT('',(-9.5,4.5,0.));
#12444=CARTESIAN_POINT('',(3.5,4.5,0.));
#12445=CARTESIAN_POINT('',(-9.5,4.5,1.));
#12446=CARTESIAN_POINT('',(-9.5,4.5,0.));
#12447=CARTESIAN_POINT('',(3.5,4.5,1.));
#12448=CARTESIAN_POINT('',(3.5,4.5,1.));
#12449=CARTESIAN_POINT('',(3.5,4.5,0.));
#12450=CARTESIAN_POINT('Origin',(3.5,-7.,0.));
#12451=CARTESIAN_POINT('',(3.5,-7.,0.));
#12452=CARTESIAN_POINT('',(3.5,-7.,0.));
#12453=CARTESIAN_POINT('',(3.5,-7.,1.));
#12454=CARTESIAN_POINT('',(3.5,-7.,1.));
#12455=CARTESIAN_POINT('',(3.5,-7.,0.));
#12456=CARTESIAN_POINT('Origin',(-9.5,-7.,0.));
#12457=CARTESIAN_POINT('',(-9.5,-7.,0.));
#12458=CARTESIAN_POINT('',(-9.5,-7.,0.));
#12459=CARTESIAN_POINT('',(-9.5,-7.,1.));
#12460=CARTESIAN_POINT('',(-9.5,-7.,1.));
#12461=CARTESIAN_POINT('',(-9.5,-7.,0.));
#12462=CARTESIAN_POINT('Origin',(-9.5,4.5,0.));
#12463=CARTESIAN_POINT('',(-9.5,4.5,0.));
#12464=CARTESIAN_POINT('',(-9.5,4.5,1.));
#12465=CARTESIAN_POINT('Origin',(-3.,-1.25,1.));
#12466=CARTESIAN_POINT('Origin',(-3.,-1.25,0.));
#15115=UNCERTAINTY_MEASURE_WITH_UNIT(LENGTH_MEASURE(0.001),#15213,
'DISTANCE_ACCURACY_VALUE',
'Maximum model space distance between geometric entities at asserted c
onnectivities');
#15162=UNCERTAINTY_MEASURE_WITH_UNIT(LENGTH_MEASURE(0.001),#15213,
'DISTANCE_ACCURACY_VALUE',
'Maximum model space distance between geometric entities at asserted c
onnectivities');
#15165=(
GEOMETRIC_REPRESENTATION_CONTEXT(3)
GLOBAL_UNCERTAINTY_ASSIGNED_CONTEXT((#15115))
GLOBAL_UNIT_ASSIGNED_CONTEXT((#15213,#15215,#15216))
REPRESENTATION_CONTEXT('','3D')
);
#15212=(
GEOMETRIC_REPRESENTATION_CONTEXT(3)
GLOBAL_UNCERTAINTY_ASSIGNED_CONTEXT((#15162))
GLOBAL_UNIT_ASSIGNED_CONTEXT((#15213,#15215,#15216))
REPRESENTATION_CONTEXT('','3D')
);
#15213=(
LENGTH_UNIT()
NAMED_UNIT(*)
SI_UNIT(.CENTI.,.METRE.)
);
#15215=(
NAMED_UNIT(*)
PLANE_ANGLE_UNIT()
SI_UNIT($,.RADIAN.)
);
#15216=(
NAMED_UNIT(*)
SI_UNIT($,.STERADIAN.)
SOLID_ANGLE_UNIT()
);
#15219=SHAPE_DEFINITION_REPRESENTATION(#15268,#15403);
#15268=PRODUCT_DEFINITION_SHAPE('',$,#15453);
#15403=SHAPE_REPRESENTATION('',(#8765),#15165);
#15450=PRODUCT_DEFINITION_CONTEXT('part definition',#15599,'design');
#15453=PRODUCT_DEFINITION('Base','Base',#15502,#15450);
#15502=PRODUCT_DEFINITION_FORMATION('',$,#15603);
#15599=APPLICATION_CONTEXT(
'Core Data for Automotive Mechanical Design Process');
#15600=PRODUCT_CONTEXT('part definition',#15599,'mechanical');
#15603=PRODUCT('Base','Base','Base',(#15600));
#15692=COLOUR_RGB('Dark Blue',0.08,0.2,0.34);
#15693=FILL_AREA_STYLE_COLOUR('',#15692);
#15694=FILL_AREA_STYLE('',(#15693));
#15695=SURFACE_STYLE_FILL_AREA(#15694);
#15696=SURFACE_SIDE_STYLE('',(#15695));
#15697=SURFACE_STYLE_USAGE(.BOTH.,#15696);
#15698=PRESENTATION_STYLE_ASSIGNMENT((#15697));
ENDSEC;
END-ISO-10303-21;
